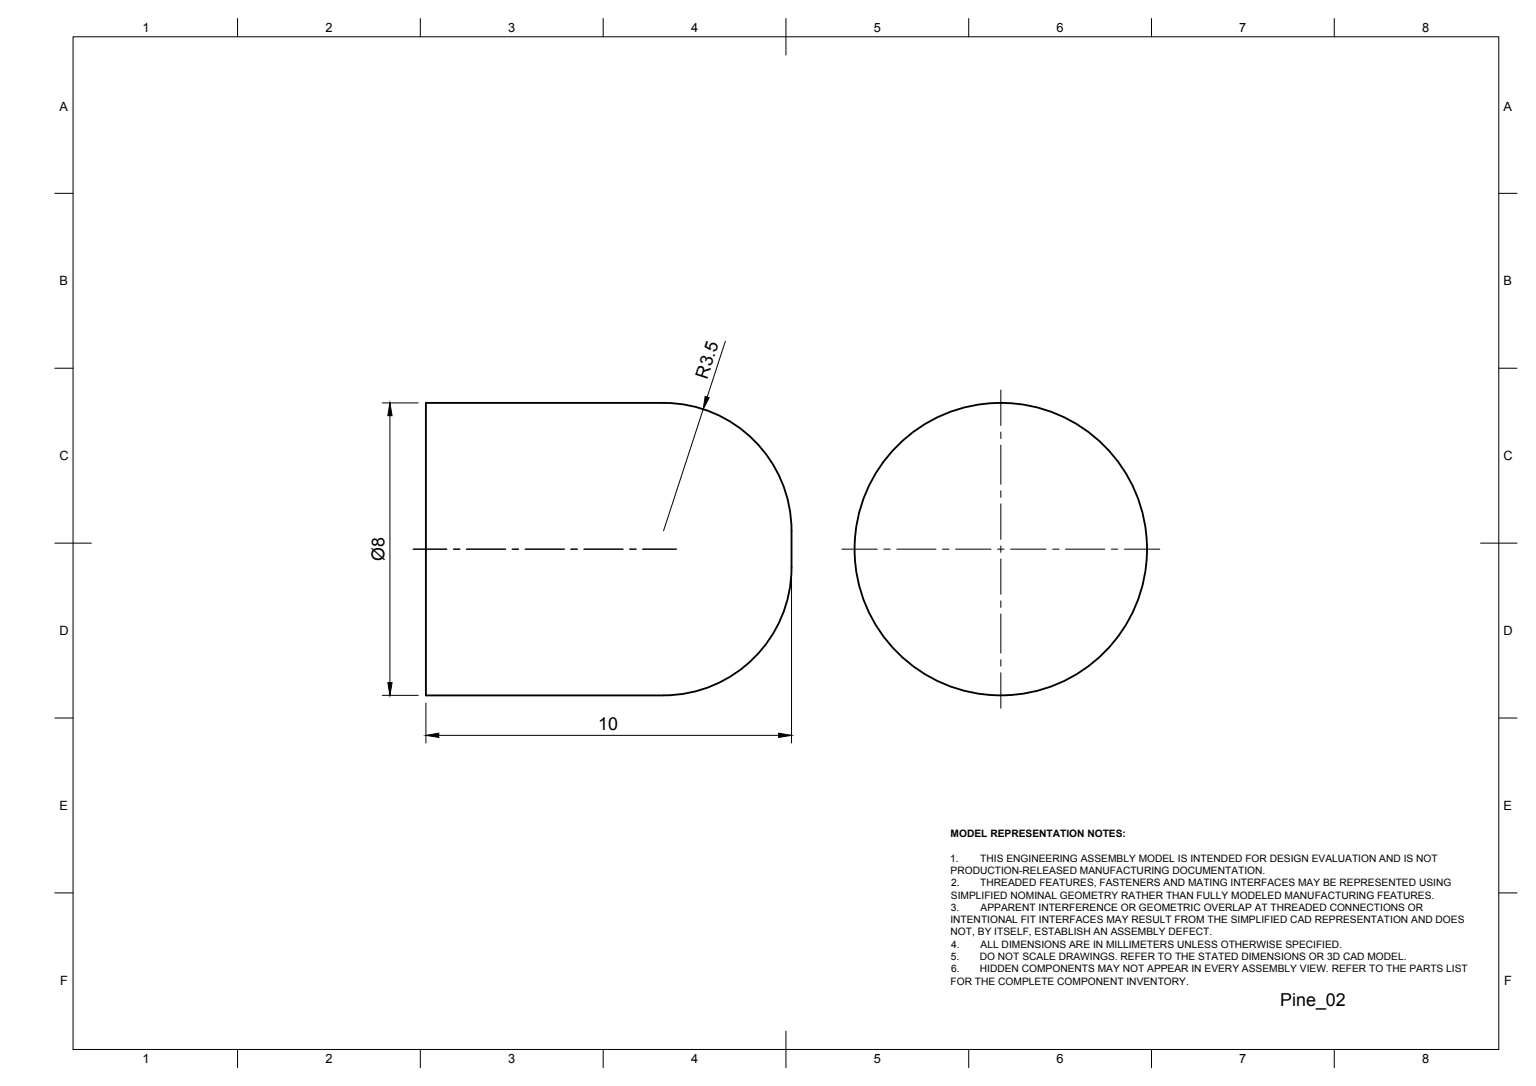
ISO-10303-21;
HEADER;
/* Generated by software containing ST-Developer
 * from STEP Tools, Inc. (www.steptools.com) 
 */

FILE_DESCRIPTION(
/* description */ (''),
/* implementation_level */ '2;1');

FILE_NAME(
/* name */ 'Pine_02.step',
/* time_stamp */ '2026-10-06T13:31:15-07:00',
/* author */ (''),
/* organization */ (''),
/* preprocessor_version */ 'ST-DEVELOPER v20.2',
/* originating_system */ 'Autodesk Translation Framework v15.15.0.0',
/* authorisation */ '');

FILE_SCHEMA (('AUTOMOTIVE_DESIGN { 1 0 10303 214 3 1 1 }'));
ENDSEC;

DATA;
#10=MECHANICAL_DESIGN_GEOMETRIC_PRESENTATION_REPRESENTATION('',(#83),#3154);
#48=(
BOUNDED_SURFACE()
B_SPLINE_SURFACE(2,2,((#2183,#2184,#2185,#2186,#2187,#2188,#2189,#2190,
#2191),(#2192,#2193,#2194,#2195,#2196,#2197,#2198,#2199,#2200),(#2201,#2202,
#2203,#2204,#2205,#2206,#2207,#2208,#2209)),.UNSPECIFIED.,.F.,.T.,.F.)
B_SPLINE_SURFACE_WITH_KNOTS((3,3),(3,2,2,2,3),(-1.57079632679509,1.96675441490332E-13),
(-3.14159265358979,-1.5707963267949,0.,1.5707963267949,3.14159265358979),
 .UNSPECIFIED.)
GEOMETRIC_REPRESENTATION_ITEM()
RATIONAL_B_SPLINE_SURFACE(((1.,0.707106781186548,1.,0.707106781186548,1.,
0.707106781186548,1.,0.707106781186548,1.),(0.707106781186405,0.499999999999899,
0.707106781186405,0.499999999999899,0.707106781186405,0.499999999999899,
0.707106781186405,0.499999999999899,0.707106781186405),(1.,0.707106781186548,
1.,0.707106781186548,1.,0.707106781186548,1.,0.707106781186548,1.)))
REPRESENTATION_ITEM('')
SURFACE()
);
#65=SHAPE_REPRESENTATION_RELATIONSHIP('SRR','None',#3193,#74);
#74=ADVANCED_BREP_SHAPE_REPRESENTATION('',(#92),#3149);
#83=STYLED_ITEM('',(#3243),#92);
#92=MANIFOLD_SOLID_BREP('Body1',#1085);
#112=PLANE('',#1237);
#113=PLANE('',#1238);
#152=CIRCLE('',#1231,3.99999999999999);
#153=CIRCLE('',#1232,3.99999999999999);
#154=CIRCLE('',#1233,3.49999999999994);
#155=CIRCLE('',#1234,0.49999999999999);
#156=CIRCLE('',#1236,3.99999999999999);
#198=FACE_OUTER_BOUND('',#262,.T.);
#199=FACE_OUTER_BOUND('',#263,.T.);
#200=FACE_OUTER_BOUND('',#264,.T.);
#201=FACE_OUTER_BOUND('',#265,.T.);
#262=EDGE_LOOP('',(#844,#845,#846,#847,#848));
#263=EDGE_LOOP('',(#849,#850,#851,#852,#853));
#264=EDGE_LOOP('',(#854));
#265=EDGE_LOOP('',(#855));
#331=LINE('',#2220,#397);
#397=VECTOR('',#1411,3.99999999999999);
#520=VERTEX_POINT('',#2210);
#521=VERTEX_POINT('',#2211);
#522=VERTEX_POINT('',#2214);
#523=VERTEX_POINT('',#2218);
#638=EDGE_CURVE('',#520,#521,#152,.T.);
#639=EDGE_CURVE('',#521,#520,#153,.T.);
#640=EDGE_CURVE('',#521,#522,#154,.T.);
#641=EDGE_CURVE('',#522,#522,#155,.T.);
#642=EDGE_CURVE('',#523,#523,#156,.T.);
#643=EDGE_CURVE('',#523,#520,#331,.T.);
#844=ORIENTED_EDGE('',*,*,#638,.F.);
#845=ORIENTED_EDGE('',*,*,#639,.F.);
#846=ORIENTED_EDGE('',*,*,#640,.T.);
#847=ORIENTED_EDGE('',*,*,#641,.F.);
#848=ORIENTED_EDGE('',*,*,#640,.F.);
#849=ORIENTED_EDGE('',*,*,#642,.F.);
#850=ORIENTED_EDGE('',*,*,#643,.T.);
#851=ORIENTED_EDGE('',*,*,#638,.T.);
#852=ORIENTED_EDGE('',*,*,#639,.T.);
#853=ORIENTED_EDGE('',*,*,#643,.F.);
#854=ORIENTED_EDGE('',*,*,#641,.T.);
#855=ORIENTED_EDGE('',*,*,#642,.T.);
#1015=CYLINDRICAL_SURFACE('',#1235,3.99999999999999);
#1049=ADVANCED_FACE('',(#198),#48,.F.);
#1050=ADVANCED_FACE('',(#199),#1015,.T.);
#1051=ADVANCED_FACE('',(#200),#112,.F.);
#1052=ADVANCED_FACE('',(#201),#113,.T.);
#1085=CLOSED_SHELL('',(#1049,#1050,#1051,#1052));
#1230=AXIS2_PLACEMENT_3D('',#2182,#1397,#1398);
#1231=AXIS2_PLACEMENT_3D('',#2212,#1399,#1400);
#1232=AXIS2_PLACEMENT_3D('',#2213,#1401,#1402);
#1233=AXIS2_PLACEMENT_3D('',#2215,#1403,#1404);
#1234=AXIS2_PLACEMENT_3D('',#2216,#1405,#1406);
#1235=AXIS2_PLACEMENT_3D('',#2217,#1407,#1408);
#1236=AXIS2_PLACEMENT_3D('',#2219,#1409,#1410);
#1237=AXIS2_PLACEMENT_3D('',#2221,#1412,#1413);
#1238=AXIS2_PLACEMENT_3D('',#2222,#1414,#1415);
#1397=DIRECTION('axis',(0.,0.,1.));
#1398=DIRECTION('refdir',(1.,0.,0.));
#1399=DIRECTION('center_axis',(1.,0.,0.));
#1400=DIRECTION('ref_axis',(0.,1.,0.));
#1401=DIRECTION('center_axis',(1.,0.,0.));
#1402=DIRECTION('ref_axis',(0.,1.,0.));
#1403=DIRECTION('center_axis',(-3.42164774028179E-14,-1.,-1.22464679909721E-16));
#1404=DIRECTION('ref_axis',(1.46549439250521E-13,-1.22464679914735E-16,
1.));
#1405=DIRECTION('center_axis',(-1.,0.,0.));
#1406=DIRECTION('ref_axis',(0.,1.,0.));
#1407=DIRECTION('center_axis',(1.,0.,0.));
#1408=DIRECTION('ref_axis',(0.,1.,0.));
#1409=DIRECTION('center_axis',(1.,0.,0.));
#1410=DIRECTION('ref_axis',(0.,1.,0.));
#1411=DIRECTION('',(-1.,0.,0.));
#1412=DIRECTION('center_axis',(1.,0.,0.));
#1413=DIRECTION('ref_axis',(0.,1.,0.));
#1414=DIRECTION('center_axis',(1.,0.,0.));
#1415=DIRECTION('ref_axis',(0.,1.,0.));
#2182=CARTESIAN_POINT('',(0.,0.,0.));
#2183=CARTESIAN_POINT('Ctrl Pts',(-24.9999999999999,1.38434137533096E-13,
180.5));
#2184=CARTESIAN_POINT('Ctrl Pts',(-24.9999999999999,-0.499999999999194,
180.5));
#2185=CARTESIAN_POINT('Ctrl Pts',(-25.,-0.499999999999194,180.000000000001));
#2186=CARTESIAN_POINT('Ctrl Pts',(-25.0000000000001,-0.499999999999194,
179.500000000001));
#2187=CARTESIAN_POINT('Ctrl Pts',(-25.0000000000001,1.38434137533096E-13,
179.500000000001));
#2188=CARTESIAN_POINT('Ctrl Pts',(-25.0000000000001,0.49999999999947,179.500000000001));
#2189=CARTESIAN_POINT('Ctrl Pts',(-25.,0.499999999999471,180.000000000001));
#2190=CARTESIAN_POINT('Ctrl Pts',(-24.9999999999999,0.49999999999947,180.5));
#2191=CARTESIAN_POINT('Ctrl Pts',(-24.9999999999999,1.38434137533096E-13,
180.5));
#2192=CARTESIAN_POINT('Ctrl Pts',(-25.0000000000001,1.38434137533119E-13,
184.000000000001));
#2193=CARTESIAN_POINT('Ctrl Pts',(-25.0000000000002,-4.00000000000052,184.000000000001));
#2194=CARTESIAN_POINT('Ctrl Pts',(-25.0000000000008,-4.00000000000052,180.000000000001));
#2195=CARTESIAN_POINT('Ctrl Pts',(-25.0000000000014,-4.00000000000052,176.));
#2196=CARTESIAN_POINT('Ctrl Pts',(-25.0000000000013,1.38434137533119E-13,
176.));
#2197=CARTESIAN_POINT('Ctrl Pts',(-25.0000000000011,4.0000000000008,176.));
#2198=CARTESIAN_POINT('Ctrl Pts',(-25.0000000000005,4.0000000000008,180.000000000001));
#2199=CARTESIAN_POINT('Ctrl Pts',(-25.,4.0000000000008,184.000000000001));
#2200=CARTESIAN_POINT('Ctrl Pts',(-25.0000000000001,1.38434137533119E-13,
184.000000000001));
#2201=CARTESIAN_POINT('Ctrl Pts',(-21.4999999999988,1.86764666232119E-14,
184.));
#2202=CARTESIAN_POINT('Ctrl Pts',(-21.4999999999989,-3.99999999999997,184.));
#2203=CARTESIAN_POINT('Ctrl Pts',(-21.4999999999995,-3.99999999999997,180.));
#2204=CARTESIAN_POINT('Ctrl Pts',(-21.5000000000001,-3.99999999999997,176.));
#2205=CARTESIAN_POINT('Ctrl Pts',(-21.5,1.86764666232117E-14,176.));
#2206=CARTESIAN_POINT('Ctrl Pts',(-21.4999999999998,4.,176.));
#2207=CARTESIAN_POINT('Ctrl Pts',(-21.4999999999992,4.,180.));
#2208=CARTESIAN_POINT('Ctrl Pts',(-21.4999999999986,4.,184.));
#2209=CARTESIAN_POINT('Ctrl Pts',(-21.4999999999988,1.86764666232119E-14,
184.));
#2210=CARTESIAN_POINT('',(-21.5,-3.99999999999999,180.));
#2211=CARTESIAN_POINT('',(-21.5,1.81866079035945E-14,184.));
#2212=CARTESIAN_POINT('Origin',(-21.5,0.,180.));
#2213=CARTESIAN_POINT('Origin',(-21.5,0.,180.));
#2214=CARTESIAN_POINT('',(-25.,-6.12323399573644E-17,180.5));
#2215=CARTESIAN_POINT('Origin',(-21.5,1.86152342832779E-14,180.5));
#2216=CARTESIAN_POINT('Origin',(-25.,0.,180.));
#2217=CARTESIAN_POINT('Origin',(0.,0.,180.));
#2218=CARTESIAN_POINT('',(-15.,-3.99999999999999,180.));
#2219=CARTESIAN_POINT('Origin',(-15.,0.,180.));
#2220=CARTESIAN_POINT('',(0.,-3.99999999999999,180.));
#2221=CARTESIAN_POINT('Origin',(-25.,0.,180.));
#2222=CARTESIAN_POINT('Origin',(-15.,0.,180.));
#3138=UNCERTAINTY_MEASURE_WITH_UNIT(LENGTH_MEASURE(0.01),#3155,
'DISTANCE_ACCURACY_VALUE',
'Maximum model space distance between geometric entities at asserted c
onnectivities');
#3143=UNCERTAINTY_MEASURE_WITH_UNIT(LENGTH_MEASURE(0.01),#3155,
'DISTANCE_ACCURACY_VALUE',
'Maximum model space distance between geometric entities at asserted c
onnectivities');
#3149=(
GEOMETRIC_REPRESENTATION_CONTEXT(3)
GLOBAL_UNCERTAINTY_ASSIGNED_CONTEXT((#3138))
GLOBAL_UNIT_ASSIGNED_CONTEXT((#3155,#3157,#3158))
REPRESENTATION_CONTEXT('','3D')
);
#3154=(
GEOMETRIC_REPRESENTATION_CONTEXT(3)
GLOBAL_UNCERTAINTY_ASSIGNED_CONTEXT((#3143))
GLOBAL_UNIT_ASSIGNED_CONTEXT((#3155,#3157,#3158))
REPRESENTATION_CONTEXT('','3D')
);
#3155=(
LENGTH_UNIT()
NAMED_UNIT(*)
SI_UNIT(.MILLI.,.METRE.)
);
#3157=(
NAMED_UNIT(*)
PLANE_ANGLE_UNIT()
SI_UNIT($,.RADIAN.)
);
#3158=(
NAMED_UNIT(*)
SI_UNIT($,.STERADIAN.)
SOLID_ANGLE_UNIT()
);
#3164=SHAPE_DEFINITION_REPRESENTATION(#3174,#3193);
#3174=PRODUCT_DEFINITION_SHAPE('',$,#3204);
#3193=SHAPE_REPRESENTATION('',(#1230),#3149);
#3198=PRODUCT_DEFINITION_CONTEXT('part definition',#3230,'design');
#3204=PRODUCT_DEFINITION('Pine_02','Pine_02',#3214,#3198);
#3214=PRODUCT_DEFINITION_FORMATION('',$,#3237);
#3230=APPLICATION_CONTEXT(
'Core Data for Automotive Mechanical Design Process');
#3231=PRODUCT_CONTEXT('part definition',#3230,'mechanical');
#3237=PRODUCT('Pine_02','Pine_02',$,(#3231));
#3243=PRESENTATION_STYLE_ASSIGNMENT((#3245));
#3245=SURFACE_STYLE_USAGE(.BOTH.,#3247);
#3247=SURFACE_SIDE_STYLE('',(#3249));
#3249=SURFACE_STYLE_FILL_AREA(#3251);
#3251=FILL_AREA_STYLE('Opaque(160,160,160)',(#3253));
#3253=FILL_AREA_STYLE_COLOUR('Opaque(160,160,160)',#3255);
#3255=COLOUR_RGB('Opaque(160,160,160)', 0.09019608, 0.27058824, 0.51372549);
ENDSEC;
END-ISO-10303-21;
